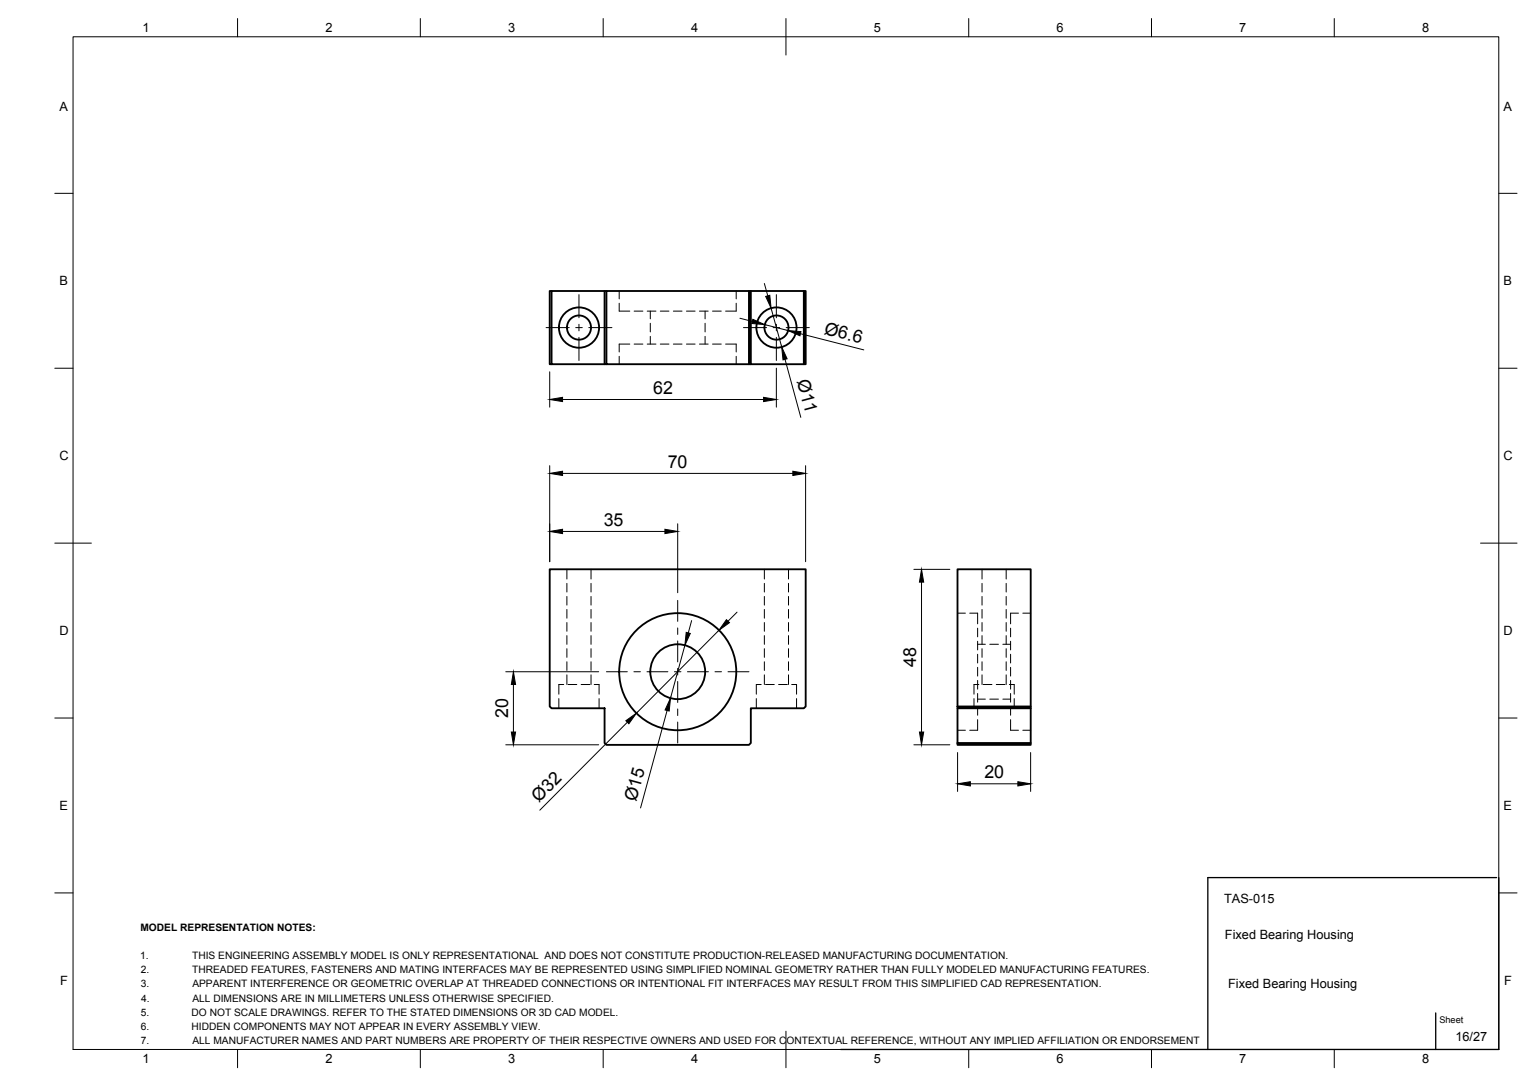
ISO-10303-21;
HEADER;
/* Generated by software containing ST-Developer
 * from STEP Tools, Inc. (www.steptools.com) 
 */

FILE_DESCRIPTION(
/* description */ ('STEP AP214'),
/* implementation_level */ '2;1');

FILE_NAME(
/* name */ 'Fixed Bearing Housing.step',
/* time_stamp */ '2026-11-15T14:49:54-08:00',
/* author */ (''),
/* organization */ (''),
/* preprocessor_version */ 'ST-DEVELOPER v20.2',
/* originating_system */ 'Autodesk Translation Framework v15.17.0.0',
/* authorisation */ '');

FILE_SCHEMA (('AUTOMOTIVE_DESIGN { 1 0 10303 214 3 1 1 }'));
ENDSEC;

DATA;
#10=MECHANICAL_DESIGN_GEOMETRIC_PRESENTATION_REPRESENTATION('',(#1109),#66721);
#1047=SHAPE_REPRESENTATION_RELATIONSHIP('SRR','None',#66907,#1078);
#1078=ADVANCED_BREP_SHAPE_REPRESENTATION('',(#1144),#66698);
#1109=STYLED_ITEM('',(#67095),#1144);
#1144=MANIFOLD_SOLID_BREP('Body1',#25675);
#1328=FACE_BOUND('',#4545,.T.);
#1329=FACE_BOUND('',#4549,.T.);
#1330=FACE_BOUND('',#4550,.T.);
#1331=FACE_BOUND('',#4554,.T.);
#1332=FACE_BOUND('',#4561,.T.);
#1333=FACE_BOUND('',#4563,.T.);
#1334=FACE_BOUND('',#4565,.T.);
#1335=FACE_BOUND('',#4567,.T.);
#1336=FACE_BOUND('',#4569,.T.);
#1337=FACE_BOUND('',#4571,.T.);
#1889=PLANE('',#27417);
#1890=PLANE('',#27418);
#1891=PLANE('',#27419);
#1892=PLANE('',#27420);
#1893=PLANE('',#27421);
#1894=PLANE('',#27422);
#1895=PLANE('',#27423);
#1896=PLANE('',#27424);
#1897=PLANE('',#27425);
#1898=PLANE('',#27426);
#1899=PLANE('',#27427);
#1900=PLANE('',#27428);
#1901=PLANE('',#27429);
#1902=PLANE('',#27430);
#1903=PLANE('',#27431);
#1904=PLANE('',#27432);
#1905=PLANE('',#27433);
#1906=PLANE('',#27434);
#2935=FACE_OUTER_BOUND('',#4537,.T.);
#2936=FACE_OUTER_BOUND('',#4538,.T.);
#2937=FACE_OUTER_BOUND('',#4539,.T.);
#2938=FACE_OUTER_BOUND('',#4540,.T.);
#2939=FACE_OUTER_BOUND('',#4541,.T.);
#2940=FACE_OUTER_BOUND('',#4542,.T.);
#2941=FACE_OUTER_BOUND('',#4543,.T.);
#2942=FACE_OUTER_BOUND('',#4544,.T.);
#2943=FACE_OUTER_BOUND('',#4546,.T.);
#2944=FACE_OUTER_BOUND('',#4547,.T.);
#2945=FACE_OUTER_BOUND('',#4548,.T.);
#2946=FACE_OUTER_BOUND('',#4551,.T.);
#2947=FACE_OUTER_BOUND('',#4552,.T.);
#2948=FACE_OUTER_BOUND('',#4553,.T.);
#2949=FACE_OUTER_BOUND('',#4555,.T.);
#2950=FACE_OUTER_BOUND('',#4556,.T.);
#2951=FACE_OUTER_BOUND('',#4557,.T.);
#2952=FACE_OUTER_BOUND('',#4558,.T.);
#2953=FACE_OUTER_BOUND('',#4559,.T.);
#2954=FACE_OUTER_BOUND('',#4560,.T.);
#2955=FACE_OUTER_BOUND('',#4562,.T.);
#2956=FACE_OUTER_BOUND('',#4564,.T.);
#2957=FACE_OUTER_BOUND('',#4566,.T.);
#2958=FACE_OUTER_BOUND('',#4568,.T.);
#2959=FACE_OUTER_BOUND('',#4570,.T.);
#4537=EDGE_LOOP('',(#20216,#20217,#20218,#20219));
#4538=EDGE_LOOP('',(#20220,#20221,#20222,#20223));
#4539=EDGE_LOOP('',(#20224,#20225,#20226,#20227));
#4540=EDGE_LOOP('',(#20228,#20229,#20230,#20231));
#4541=EDGE_LOOP('',(#20232,#20233,#20234,#20235));
#4542=EDGE_LOOP('',(#20236,#20237,#20238,#20239));
#4543=EDGE_LOOP('',(#20240,#20241,#20242,#20243));
#4544=EDGE_LOOP('',(#20244,#20245,#20246,#20247));
#4545=EDGE_LOOP('',(#20248));
#4546=EDGE_LOOP('',(#20249,#20250,#20251,#20252));
#4547=EDGE_LOOP('',(#20253,#20254,#20255,#20256));
#4548=EDGE_LOOP('',(#20257,#20258,#20259,#20260));
#4549=EDGE_LOOP('',(#20261));
#4550=EDGE_LOOP('',(#20262));
#4551=EDGE_LOOP('',(#20263,#20264,#20265,#20266));
#4552=EDGE_LOOP('',(#20267,#20268,#20269,#20270));
#4553=EDGE_LOOP('',(#20271,#20272,#20273,#20274));
#4554=EDGE_LOOP('',(#20275));
#4555=EDGE_LOOP('',(#20276,#20277,#20278,#20279));
#4556=EDGE_LOOP('',(#20280,#20281,#20282,#20283));
#4557=EDGE_LOOP('',(#20284,#20285,#20286,#20287));
#4558=EDGE_LOOP('',(#20288,#20289,#20290,#20291));
#4559=EDGE_LOOP('',(#20292,#20293,#20294,#20295));
#4560=EDGE_LOOP('',(#20296,#20297,#20298,#20299,#20300,#20301,#20302,#20303,
#20304,#20305,#20306,#20307));
#4561=EDGE_LOOP('',(#20308));
#4562=EDGE_LOOP('',(#20309,#20310,#20311,#20312,#20313,#20314,#20315,#20316,
#20317,#20318,#20319,#20320));
#4563=EDGE_LOOP('',(#20321));
#4564=EDGE_LOOP('',(#20322));
#4565=EDGE_LOOP('',(#20323));
#4566=EDGE_LOOP('',(#20324));
#4567=EDGE_LOOP('',(#20325));
#4568=EDGE_LOOP('',(#20326));
#4569=EDGE_LOOP('',(#20327));
#4570=EDGE_LOOP('',(#20328));
#4571=EDGE_LOOP('',(#20329));
#6589=LINE('',#40218,#8578);
#6590=LINE('',#40224,#8579);
#6591=LINE('',#40230,#8580);
#6592=LINE('',#40236,#8581);
#6593=LINE('',#40242,#8582);
#6594=LINE('',#40248,#8583);
#6595=LINE('',#40254,#8584);
#6596=LINE('',#40259,#8585);
#6597=LINE('',#40261,#8586);
#6598=LINE('',#40263,#8587);
#6599=LINE('',#40264,#8588);
#6600=LINE('',#40267,#8589);
#6601=LINE('',#40269,#8590);
#6602=LINE('',#40270,#8591);
#6603=LINE('',#40273,#8592);
#6604=LINE('',#40275,#8593);
#6605=LINE('',#40276,#8594);
#6606=LINE('',#40279,#8595);
#6607=LINE('',#40281,#8596);
#6608=LINE('',#40282,#8597);
#6609=LINE('',#40285,#8598);
#6610=LINE('',#40287,#8599);
#6611=LINE('',#40288,#8600);
#6612=LINE('',#40291,#8601);
#6613=LINE('',#40293,#8602);
#6614=LINE('',#40294,#8603);
#6615=LINE('',#40297,#8604);
#6616=LINE('',#40299,#8605);
#6617=LINE('',#40300,#8606);
#6618=LINE('',#40303,#8607);
#6619=LINE('',#40305,#8608);
#6620=LINE('',#40306,#8609);
#6621=LINE('',#40309,#8610);
#6622=LINE('',#40311,#8611);
#6623=LINE('',#40312,#8612);
#6624=LINE('',#40315,#8613);
#6625=LINE('',#40317,#8614);
#6626=LINE('',#40318,#8615);
#6627=LINE('',#40321,#8616);
#6628=LINE('',#40323,#8617);
#6629=LINE('',#40324,#8618);
#6630=LINE('',#40326,#8619);
#6631=LINE('',#40327,#8620);
#8578=VECTOR('',#32576,16.);
#8579=VECTOR('',#32583,7.5);
#8580=VECTOR('',#32590,16.);
#8581=VECTOR('',#32597,5.5);
#8582=VECTOR('',#32604,3.3);
#8583=VECTOR('',#32611,5.5);
#8584=VECTOR('',#32618,3.3);
#8585=VECTOR('',#32623,1000.);
#8586=VECTOR('',#32624,1000.);
#8587=VECTOR('',#32625,1000.);
#8588=VECTOR('',#32626,1000.);
#8589=VECTOR('',#32629,1000.);
#8590=VECTOR('',#32630,1000.);
#8591=VECTOR('',#32631,1000.);
#8592=VECTOR('',#32634,1000.);
#8593=VECTOR('',#32635,1000.);
#8594=VECTOR('',#32636,1000.);
#8595=VECTOR('',#32639,1000.);
#8596=VECTOR('',#32640,1000.);
#8597=VECTOR('',#32641,1000.);
#8598=VECTOR('',#32644,1000.);
#8599=VECTOR('',#32645,1000.);
#8600=VECTOR('',#32646,1000.);
#8601=VECTOR('',#32649,1000.);
#8602=VECTOR('',#32650,1000.);
#8603=VECTOR('',#32651,1000.);
#8604=VECTOR('',#32654,1000.);
#8605=VECTOR('',#32655,1000.);
#8606=VECTOR('',#32656,1000.);
#8607=VECTOR('',#32659,1000.);
#8608=VECTOR('',#32660,1000.);
#8609=VECTOR('',#32661,1000.);
#8610=VECTOR('',#32664,1000.);
#8611=VECTOR('',#32665,1000.);
#8612=VECTOR('',#32666,1000.);
#8613=VECTOR('',#32669,1000.);
#8614=VECTOR('',#32670,1000.);
#8615=VECTOR('',#32671,1000.);
#8616=VECTOR('',#32674,1000.);
#8617=VECTOR('',#32675,1000.);
#8618=VECTOR('',#32676,1000.);
#8619=VECTOR('',#32679,1000.);
#8620=VECTOR('',#32680,1000.);
#10044=CIRCLE('',#27397,16.);
#10045=CIRCLE('',#27398,16.);
#10046=CIRCLE('',#27400,7.5);
#10047=CIRCLE('',#27401,7.5);
#10048=CIRCLE('',#27403,16.);
#10049=CIRCLE('',#27404,16.);
#10050=CIRCLE('',#27406,5.5);
#10051=CIRCLE('',#27407,5.5);
#10052=CIRCLE('',#27409,3.29999999999999);
#10053=CIRCLE('',#27410,3.3);
#10054=CIRCLE('',#27412,5.5);
#10055=CIRCLE('',#27413,5.5);
#10056=CIRCLE('',#27415,3.29999999999999);
#10057=CIRCLE('',#27416,3.3);
#11835=VERTEX_POINT('',#40215);
#11836=VERTEX_POINT('',#40217);
#11837=VERTEX_POINT('',#40221);
#11838=VERTEX_POINT('',#40223);
#11839=VERTEX_POINT('',#40227);
#11840=VERTEX_POINT('',#40229);
#11841=VERTEX_POINT('',#40233);
#11842=VERTEX_POINT('',#40235);
#11843=VERTEX_POINT('',#40239);
#11844=VERTEX_POINT('',#40241);
#11845=VERTEX_POINT('',#40245);
#11846=VERTEX_POINT('',#40247);
#11847=VERTEX_POINT('',#40251);
#11848=VERTEX_POINT('',#40253);
#11849=VERTEX_POINT('',#40257);
#11850=VERTEX_POINT('',#40258);
#11851=VERTEX_POINT('',#40260);
#11852=VERTEX_POINT('',#40262);
#11853=VERTEX_POINT('',#40266);
#11854=VERTEX_POINT('',#40268);
#11855=VERTEX_POINT('',#40272);
#11856=VERTEX_POINT('',#40274);
#11857=VERTEX_POINT('',#40278);
#11858=VERTEX_POINT('',#40280);
#11859=VERTEX_POINT('',#40284);
#11860=VERTEX_POINT('',#40286);
#11861=VERTEX_POINT('',#40290);
#11862=VERTEX_POINT('',#40292);
#11863=VERTEX_POINT('',#40296);
#11864=VERTEX_POINT('',#40298);
#11865=VERTEX_POINT('',#40302);
#11866=VERTEX_POINT('',#40304);
#11867=VERTEX_POINT('',#40308);
#11868=VERTEX_POINT('',#40310);
#11869=VERTEX_POINT('',#40314);
#11870=VERTEX_POINT('',#40316);
#11871=VERTEX_POINT('',#40320);
#11872=VERTEX_POINT('',#40322);
#14801=EDGE_CURVE('',#11835,#11835,#10044,.T.);
#14802=EDGE_CURVE('',#11835,#11836,#6589,.T.);
#14803=EDGE_CURVE('',#11836,#11836,#10045,.T.);
#14804=EDGE_CURVE('',#11837,#11837,#10046,.T.);
#14805=EDGE_CURVE('',#11837,#11838,#6590,.T.);
#14806=EDGE_CURVE('',#11838,#11838,#10047,.T.);
#14807=EDGE_CURVE('',#11839,#11839,#10048,.T.);
#14808=EDGE_CURVE('',#11839,#11840,#6591,.T.);
#14809=EDGE_CURVE('',#11840,#11840,#10049,.T.);
#14810=EDGE_CURVE('',#11841,#11841,#10050,.T.);
#14811=EDGE_CURVE('',#11841,#11842,#6592,.T.);
#14812=EDGE_CURVE('',#11842,#11842,#10051,.T.);
#14813=EDGE_CURVE('',#11843,#11843,#10052,.T.);
#14814=EDGE_CURVE('',#11843,#11844,#6593,.T.);
#14815=EDGE_CURVE('',#11844,#11844,#10053,.T.);
#14816=EDGE_CURVE('',#11845,#11845,#10054,.T.);
#14817=EDGE_CURVE('',#11845,#11846,#6594,.T.);
#14818=EDGE_CURVE('',#11846,#11846,#10055,.T.);
#14819=EDGE_CURVE('',#11847,#11847,#10056,.T.);
#14820=EDGE_CURVE('',#11847,#11848,#6595,.T.);
#14821=EDGE_CURVE('',#11848,#11848,#10057,.T.);
#14822=EDGE_CURVE('',#11849,#11850,#6596,.T.);
#14823=EDGE_CURVE('',#11851,#11850,#6597,.T.);
#14824=EDGE_CURVE('',#11852,#11851,#6598,.T.);
#14825=EDGE_CURVE('',#11852,#11849,#6599,.T.);
#14826=EDGE_CURVE('',#11850,#11853,#6600,.T.);
#14827=EDGE_CURVE('',#11854,#11853,#6601,.T.);
#14828=EDGE_CURVE('',#11851,#11854,#6602,.T.);
#14829=EDGE_CURVE('',#11853,#11855,#6603,.T.);
#14830=EDGE_CURVE('',#11856,#11855,#6604,.T.);
#14831=EDGE_CURVE('',#11854,#11856,#6605,.T.);
#14832=EDGE_CURVE('',#11855,#11857,#6606,.T.);
#14833=EDGE_CURVE('',#11858,#11857,#6607,.T.);
#14834=EDGE_CURVE('',#11856,#11858,#6608,.T.);
#14835=EDGE_CURVE('',#11857,#11859,#6609,.T.);
#14836=EDGE_CURVE('',#11860,#11859,#6610,.T.);
#14837=EDGE_CURVE('',#11858,#11860,#6611,.T.);
#14838=EDGE_CURVE('',#11859,#11861,#6612,.T.);
#14839=EDGE_CURVE('',#11862,#11861,#6613,.T.);
#14840=EDGE_CURVE('',#11860,#11862,#6614,.T.);
#14841=EDGE_CURVE('',#11861,#11863,#6615,.T.);
#14842=EDGE_CURVE('',#11864,#11863,#6616,.T.);
#14843=EDGE_CURVE('',#11862,#11864,#6617,.T.);
#14844=EDGE_CURVE('',#11863,#11865,#6618,.T.);
#14845=EDGE_CURVE('',#11866,#11865,#6619,.T.);
#14846=EDGE_CURVE('',#11864,#11866,#6620,.T.);
#14847=EDGE_CURVE('',#11865,#11867,#6621,.T.);
#14848=EDGE_CURVE('',#11868,#11867,#6622,.T.);
#14849=EDGE_CURVE('',#11866,#11868,#6623,.T.);
#14850=EDGE_CURVE('',#11867,#11869,#6624,.T.);
#14851=EDGE_CURVE('',#11870,#11869,#6625,.T.);
#14852=EDGE_CURVE('',#11868,#11870,#6626,.T.);
#14853=EDGE_CURVE('',#11869,#11871,#6627,.T.);
#14854=EDGE_CURVE('',#11872,#11871,#6628,.T.);
#14855=EDGE_CURVE('',#11870,#11872,#6629,.T.);
#14856=EDGE_CURVE('',#11871,#11849,#6630,.T.);
#14857=EDGE_CURVE('',#11872,#11852,#6631,.T.);
#20216=ORIENTED_EDGE('',*,*,#14801,.F.);
#20217=ORIENTED_EDGE('',*,*,#14802,.T.);
#20218=ORIENTED_EDGE('',*,*,#14803,.T.);
#20219=ORIENTED_EDGE('',*,*,#14802,.F.);
#20220=ORIENTED_EDGE('',*,*,#14804,.F.);
#20221=ORIENTED_EDGE('',*,*,#14805,.T.);
#20222=ORIENTED_EDGE('',*,*,#14806,.T.);
#20223=ORIENTED_EDGE('',*,*,#14805,.F.);
#20224=ORIENTED_EDGE('',*,*,#14807,.F.);
#20225=ORIENTED_EDGE('',*,*,#14808,.T.);
#20226=ORIENTED_EDGE('',*,*,#14809,.T.);
#20227=ORIENTED_EDGE('',*,*,#14808,.F.);
#20228=ORIENTED_EDGE('',*,*,#14810,.F.);
#20229=ORIENTED_EDGE('',*,*,#14811,.T.);
#20230=ORIENTED_EDGE('',*,*,#14812,.T.);
#20231=ORIENTED_EDGE('',*,*,#14811,.F.);
#20232=ORIENTED_EDGE('',*,*,#14813,.F.);
#20233=ORIENTED_EDGE('',*,*,#14814,.T.);
#20234=ORIENTED_EDGE('',*,*,#14815,.T.);
#20235=ORIENTED_EDGE('',*,*,#14814,.F.);
#20236=ORIENTED_EDGE('',*,*,#14816,.F.);
#20237=ORIENTED_EDGE('',*,*,#14817,.T.);
#20238=ORIENTED_EDGE('',*,*,#14818,.T.);
#20239=ORIENTED_EDGE('',*,*,#14817,.F.);
#20240=ORIENTED_EDGE('',*,*,#14819,.F.);
#20241=ORIENTED_EDGE('',*,*,#14820,.T.);
#20242=ORIENTED_EDGE('',*,*,#14821,.T.);
#20243=ORIENTED_EDGE('',*,*,#14820,.F.);
#20244=ORIENTED_EDGE('',*,*,#14822,.T.);
#20245=ORIENTED_EDGE('',*,*,#14823,.F.);
#20246=ORIENTED_EDGE('',*,*,#14824,.F.);
#20247=ORIENTED_EDGE('',*,*,#14825,.T.);
#20248=ORIENTED_EDGE('',*,*,#14818,.F.);
#20249=ORIENTED_EDGE('',*,*,#14826,.T.);
#20250=ORIENTED_EDGE('',*,*,#14827,.F.);
#20251=ORIENTED_EDGE('',*,*,#14828,.F.);
#20252=ORIENTED_EDGE('',*,*,#14823,.T.);
#20253=ORIENTED_EDGE('',*,*,#14829,.T.);
#20254=ORIENTED_EDGE('',*,*,#14830,.F.);
#20255=ORIENTED_EDGE('',*,*,#14831,.F.);
#20256=ORIENTED_EDGE('',*,*,#14827,.T.);
#20257=ORIENTED_EDGE('',*,*,#14832,.T.);
#20258=ORIENTED_EDGE('',*,*,#14833,.F.);
#20259=ORIENTED_EDGE('',*,*,#14834,.F.);
#20260=ORIENTED_EDGE('',*,*,#14830,.T.);
#20261=ORIENTED_EDGE('',*,*,#14813,.T.);
#20262=ORIENTED_EDGE('',*,*,#14819,.T.);
#20263=ORIENTED_EDGE('',*,*,#14835,.T.);
#20264=ORIENTED_EDGE('',*,*,#14836,.F.);
#20265=ORIENTED_EDGE('',*,*,#14837,.F.);
#20266=ORIENTED_EDGE('',*,*,#14833,.T.);
#20267=ORIENTED_EDGE('',*,*,#14838,.T.);
#20268=ORIENTED_EDGE('',*,*,#14839,.F.);
#20269=ORIENTED_EDGE('',*,*,#14840,.F.);
#20270=ORIENTED_EDGE('',*,*,#14836,.T.);
#20271=ORIENTED_EDGE('',*,*,#14841,.T.);
#20272=ORIENTED_EDGE('',*,*,#14842,.F.);
#20273=ORIENTED_EDGE('',*,*,#14843,.F.);
#20274=ORIENTED_EDGE('',*,*,#14839,.T.);
#20275=ORIENTED_EDGE('',*,*,#14812,.F.);
#20276=ORIENTED_EDGE('',*,*,#14844,.T.);
#20277=ORIENTED_EDGE('',*,*,#14845,.F.);
#20278=ORIENTED_EDGE('',*,*,#14846,.F.);
#20279=ORIENTED_EDGE('',*,*,#14842,.T.);
#20280=ORIENTED_EDGE('',*,*,#14847,.T.);
#20281=ORIENTED_EDGE('',*,*,#14848,.F.);
#20282=ORIENTED_EDGE('',*,*,#14849,.F.);
#20283=ORIENTED_EDGE('',*,*,#14845,.T.);
#20284=ORIENTED_EDGE('',*,*,#14850,.T.);
#20285=ORIENTED_EDGE('',*,*,#14851,.F.);
#20286=ORIENTED_EDGE('',*,*,#14852,.F.);
#20287=ORIENTED_EDGE('',*,*,#14848,.T.);
#20288=ORIENTED_EDGE('',*,*,#14853,.T.);
#20289=ORIENTED_EDGE('',*,*,#14854,.F.);
#20290=ORIENTED_EDGE('',*,*,#14855,.F.);
#20291=ORIENTED_EDGE('',*,*,#14851,.T.);
#20292=ORIENTED_EDGE('',*,*,#14856,.T.);
#20293=ORIENTED_EDGE('',*,*,#14825,.F.);
#20294=ORIENTED_EDGE('',*,*,#14857,.F.);
#20295=ORIENTED_EDGE('',*,*,#14854,.T.);
#20296=ORIENTED_EDGE('',*,*,#14824,.T.);
#20297=ORIENTED_EDGE('',*,*,#14828,.T.);
#20298=ORIENTED_EDGE('',*,*,#14831,.T.);
#20299=ORIENTED_EDGE('',*,*,#14834,.T.);
#20300=ORIENTED_EDGE('',*,*,#14837,.T.);
#20301=ORIENTED_EDGE('',*,*,#14840,.T.);
#20302=ORIENTED_EDGE('',*,*,#14843,.T.);
#20303=ORIENTED_EDGE('',*,*,#14846,.T.);
#20304=ORIENTED_EDGE('',*,*,#14849,.T.);
#20305=ORIENTED_EDGE('',*,*,#14852,.T.);
#20306=ORIENTED_EDGE('',*,*,#14855,.T.);
#20307=ORIENTED_EDGE('',*,*,#14857,.T.);
#20308=ORIENTED_EDGE('',*,*,#14803,.F.);
#20309=ORIENTED_EDGE('',*,*,#14822,.F.);
#20310=ORIENTED_EDGE('',*,*,#14856,.F.);
#20311=ORIENTED_EDGE('',*,*,#14853,.F.);
#20312=ORIENTED_EDGE('',*,*,#14850,.F.);
#20313=ORIENTED_EDGE('',*,*,#14847,.F.);
#20314=ORIENTED_EDGE('',*,*,#14844,.F.);
#20315=ORIENTED_EDGE('',*,*,#14841,.F.);
#20316=ORIENTED_EDGE('',*,*,#14838,.F.);
#20317=ORIENTED_EDGE('',*,*,#14835,.F.);
#20318=ORIENTED_EDGE('',*,*,#14832,.F.);
#20319=ORIENTED_EDGE('',*,*,#14829,.F.);
#20320=ORIENTED_EDGE('',*,*,#14826,.F.);
#20321=ORIENTED_EDGE('',*,*,#14807,.T.);
#20322=ORIENTED_EDGE('',*,*,#14816,.T.);
#20323=ORIENTED_EDGE('',*,*,#14821,.F.);
#20324=ORIENTED_EDGE('',*,*,#14810,.T.);
#20325=ORIENTED_EDGE('',*,*,#14815,.F.);
#20326=ORIENTED_EDGE('',*,*,#14809,.F.);
#20327=ORIENTED_EDGE('',*,*,#14804,.T.);
#20328=ORIENTED_EDGE('',*,*,#14801,.T.);
#20329=ORIENTED_EDGE('',*,*,#14806,.F.);
#24042=CYLINDRICAL_SURFACE('',#27396,16.);
#24043=CYLINDRICAL_SURFACE('',#27399,7.5);
#24044=CYLINDRICAL_SURFACE('',#27402,16.);
#24045=CYLINDRICAL_SURFACE('',#27405,5.5);
#24046=CYLINDRICAL_SURFACE('',#27408,3.3);
#24047=CYLINDRICAL_SURFACE('',#27411,5.5);
#24048=CYLINDRICAL_SURFACE('',#27414,3.3);
#24888=ADVANCED_FACE('',(#2935),#24042,.F.);
#24889=ADVANCED_FACE('',(#2936),#24043,.F.);
#24890=ADVANCED_FACE('',(#2937),#24044,.F.);
#24891=ADVANCED_FACE('',(#2938),#24045,.F.);
#24892=ADVANCED_FACE('',(#2939),#24046,.F.);
#24893=ADVANCED_FACE('',(#2940),#24047,.F.);
#24894=ADVANCED_FACE('',(#2941),#24048,.F.);
#24895=ADVANCED_FACE('',(#2942,#1328),#1889,.F.);
#24896=ADVANCED_FACE('',(#2943),#1890,.F.);
#24897=ADVANCED_FACE('',(#2944),#1891,.F.);
#24898=ADVANCED_FACE('',(#2945,#1329,#1330),#1892,.F.);
#24899=ADVANCED_FACE('',(#2946),#1893,.F.);
#24900=ADVANCED_FACE('',(#2947),#1894,.F.);
#24901=ADVANCED_FACE('',(#2948,#1331),#1895,.F.);
#24902=ADVANCED_FACE('',(#2949),#1896,.F.);
#24903=ADVANCED_FACE('',(#2950),#1897,.F.);
#24904=ADVANCED_FACE('',(#2951),#1898,.F.);
#24905=ADVANCED_FACE('',(#2952),#1899,.F.);
#24906=ADVANCED_FACE('',(#2953),#1900,.F.);
#24907=ADVANCED_FACE('',(#2954,#1332),#1901,.T.);
#24908=ADVANCED_FACE('',(#2955,#1333),#1902,.F.);
#24909=ADVANCED_FACE('',(#2956,#1334),#1903,.F.);
#24910=ADVANCED_FACE('',(#2957,#1335),#1904,.F.);
#24911=ADVANCED_FACE('',(#2958,#1336),#1905,.F.);
#24912=ADVANCED_FACE('',(#2959,#1337),#1906,.F.);
#25675=CLOSED_SHELL('',(#24888,#24889,#24890,#24891,#24892,#24893,#24894,
#24895,#24896,#24897,#24898,#24899,#24900,#24901,#24902,#24903,#24904,#24905,
#24906,#24907,#24908,#24909,#24910,#24911,#24912));
#27395=AXIS2_PLACEMENT_3D('',#40213,#32570,#32571);
#27396=AXIS2_PLACEMENT_3D('',#40214,#32572,#32573);
#27397=AXIS2_PLACEMENT_3D('',#40216,#32574,#32575);
#27398=AXIS2_PLACEMENT_3D('',#40219,#32577,#32578);
#27399=AXIS2_PLACEMENT_3D('',#40220,#32579,#32580);
#27400=AXIS2_PLACEMENT_3D('',#40222,#32581,#32582);
#27401=AXIS2_PLACEMENT_3D('',#40225,#32584,#32585);
#27402=AXIS2_PLACEMENT_3D('',#40226,#32586,#32587);
#27403=AXIS2_PLACEMENT_3D('',#40228,#32588,#32589);
#27404=AXIS2_PLACEMENT_3D('',#40231,#32591,#32592);
#27405=AXIS2_PLACEMENT_3D('',#40232,#32593,#32594);
#27406=AXIS2_PLACEMENT_3D('',#40234,#32595,#32596);
#27407=AXIS2_PLACEMENT_3D('',#40237,#32598,#32599);
#27408=AXIS2_PLACEMENT_3D('',#40238,#32600,#32601);
#27409=AXIS2_PLACEMENT_3D('',#40240,#32602,#32603);
#27410=AXIS2_PLACEMENT_3D('',#40243,#32605,#32606);
#27411=AXIS2_PLACEMENT_3D('',#40244,#32607,#32608);
#27412=AXIS2_PLACEMENT_3D('',#40246,#32609,#32610);
#27413=AXIS2_PLACEMENT_3D('',#40249,#32612,#32613);
#27414=AXIS2_PLACEMENT_3D('',#40250,#32614,#32615);
#27415=AXIS2_PLACEMENT_3D('',#40252,#32616,#32617);
#27416=AXIS2_PLACEMENT_3D('',#40255,#32619,#32620);
#27417=AXIS2_PLACEMENT_3D('',#40256,#32621,#32622);
#27418=AXIS2_PLACEMENT_3D('',#40265,#32627,#32628);
#27419=AXIS2_PLACEMENT_3D('',#40271,#32632,#32633);
#27420=AXIS2_PLACEMENT_3D('',#40277,#32637,#32638);
#27421=AXIS2_PLACEMENT_3D('',#40283,#32642,#32643);
#27422=AXIS2_PLACEMENT_3D('',#40289,#32647,#32648);
#27423=AXIS2_PLACEMENT_3D('',#40295,#32652,#32653);
#27424=AXIS2_PLACEMENT_3D('',#40301,#32657,#32658);
#27425=AXIS2_PLACEMENT_3D('',#40307,#32662,#32663);
#27426=AXIS2_PLACEMENT_3D('',#40313,#32667,#32668);
#27427=AXIS2_PLACEMENT_3D('',#40319,#32672,#32673);
#27428=AXIS2_PLACEMENT_3D('',#40325,#32677,#32678);
#27429=AXIS2_PLACEMENT_3D('',#40328,#32681,#32682);
#27430=AXIS2_PLACEMENT_3D('',#40329,#32683,#32684);
#27431=AXIS2_PLACEMENT_3D('',#40330,#32685,#32686);
#27432=AXIS2_PLACEMENT_3D('',#40331,#32687,#32688);
#27433=AXIS2_PLACEMENT_3D('',#40332,#32689,#32690);
#27434=AXIS2_PLACEMENT_3D('',#40333,#32691,#32692);
#32570=DIRECTION('axis',(0.,0.,1.));
#32571=DIRECTION('refdir',(1.,0.,0.));
#32572=DIRECTION('center_axis',(1.,1.73472347597681E-16,0.));
#32573=DIRECTION('ref_axis',(-1.73472347597681E-16,1.,0.));
#32574=DIRECTION('center_axis',(1.,1.73472347597681E-16,0.));
#32575=DIRECTION('ref_axis',(-1.73472347597681E-16,1.,0.));
#32576=DIRECTION('',(1.,1.73472347597681E-16,0.));
#32577=DIRECTION('center_axis',(1.,1.73472347597681E-16,0.));
#32578=DIRECTION('ref_axis',(-1.73472347597681E-16,1.,0.));
#32579=DIRECTION('center_axis',(1.,1.73472347597681E-16,0.));
#32580=DIRECTION('ref_axis',(-1.73472347597681E-16,1.,0.));
#32581=DIRECTION('center_axis',(1.,1.73472347597681E-16,0.));
#32582=DIRECTION('ref_axis',(-1.73472347597681E-16,1.,0.));
#32583=DIRECTION('',(1.,1.73472347597681E-16,0.));
#32584=DIRECTION('center_axis',(1.,1.73472347597681E-16,0.));
#32585=DIRECTION('ref_axis',(-1.73472347597681E-16,1.,0.));
#32586=DIRECTION('center_axis',(1.,1.73472347597681E-16,0.));
#32587=DIRECTION('ref_axis',(-1.73472347597681E-16,1.,0.));
#32588=DIRECTION('center_axis',(1.,1.73472347597681E-16,0.));
#32589=DIRECTION('ref_axis',(-1.73472347597681E-16,1.,0.));
#32590=DIRECTION('',(1.,1.73472347597681E-16,0.));
#32591=DIRECTION('center_axis',(1.,1.73472347597681E-16,0.));
#32592=DIRECTION('ref_axis',(-1.73472347597681E-16,1.,0.));
#32593=DIRECTION('center_axis',(0.,1.,0.));
#32594=DIRECTION('ref_axis',(0.,0.,1.));
#32595=DIRECTION('center_axis',(0.,1.,0.));
#32596=DIRECTION('ref_axis',(0.,0.,1.));
#32597=DIRECTION('',(0.,1.,0.));
#32598=DIRECTION('center_axis',(0.,1.,0.));
#32599=DIRECTION('ref_axis',(0.,0.,1.));
#32600=DIRECTION('center_axis',(0.,1.,0.));
#32601=DIRECTION('ref_axis',(0.,0.,1.));
#32602=DIRECTION('center_axis',(0.,1.,0.));
#32603=DIRECTION('ref_axis',(0.,0.,1.));
#32604=DIRECTION('',(0.,1.,0.));
#32605=DIRECTION('center_axis',(0.,1.,0.));
#32606=DIRECTION('ref_axis',(0.,0.,1.));
#32607=DIRECTION('center_axis',(0.,1.,0.));
#32608=DIRECTION('ref_axis',(0.,0.,1.));
#32609=DIRECTION('center_axis',(0.,1.,0.));
#32610=DIRECTION('ref_axis',(0.,0.,1.));
#32611=DIRECTION('',(0.,1.,0.));
#32612=DIRECTION('center_axis',(0.,1.,0.));
#32613=DIRECTION('ref_axis',(0.,0.,1.));
#32614=DIRECTION('center_axis',(0.,1.,0.));
#32615=DIRECTION('ref_axis',(0.,0.,1.));
#32616=DIRECTION('center_axis',(0.,1.,0.));
#32617=DIRECTION('ref_axis',(0.,0.,1.));
#32618=DIRECTION('',(0.,1.,0.));
#32619=DIRECTION('center_axis',(0.,1.,0.));
#32620=DIRECTION('ref_axis',(0.,0.,1.));
#32621=DIRECTION('center_axis',(0.,-1.,-4.78544407166016E-16));
#32622=DIRECTION('ref_axis',(0.,4.78544407166016E-16,-1.));
#32623=DIRECTION('',(0.,-4.78544407166016E-16,1.));
#32624=DIRECTION('',(-1.,0.,0.));
#32625=DIRECTION('',(0.,-4.78544407166016E-16,1.));
#32626=DIRECTION('',(-1.,0.,0.));
#32627=DIRECTION('center_axis',(0.,-0.707106781186528,-0.707106781186567));
#32628=DIRECTION('ref_axis',(0.,0.707106781186567,-0.707106781186528));
#32629=DIRECTION('',(0.,-0.707106781186567,0.707106781186528));
#32630=DIRECTION('',(-1.,0.,0.));
#32631=DIRECTION('',(0.,-0.707106781186567,0.707106781186528));
#32632=DIRECTION('center_axis',(0.,3.70074341541719E-16,-1.));
#32633=DIRECTION('ref_axis',(0.,1.,3.70074341541719E-16));
#32634=DIRECTION('',(0.,-1.,-3.70074341541719E-16));
#32635=DIRECTION('',(-1.,0.,0.));
#32636=DIRECTION('',(0.,-1.,-3.70074341541719E-16));
#32637=DIRECTION('center_axis',(0.,1.,3.11362923006336E-16));
#32638=DIRECTION('ref_axis',(0.,-3.11362923006336E-16,1.));
#32639=DIRECTION('',(0.,3.11362923006336E-16,-1.));
#32640=DIRECTION('',(-1.,0.,0.));
#32641=DIRECTION('',(0.,3.11362923006336E-16,-1.));
#32642=DIRECTION('center_axis',(0.,-5.55111512312579E-16,1.));
#32643=DIRECTION('ref_axis',(0.,-1.,-5.55111512312579E-16));
#32644=DIRECTION('',(0.,1.,5.55111512312579E-16));
#32645=DIRECTION('',(-1.,0.,0.));
#32646=DIRECTION('',(0.,1.,5.55111512312579E-16));
#32647=DIRECTION('center_axis',(0.,-0.707106781186538,0.707106781186557));
#32648=DIRECTION('ref_axis',(0.,-0.707106781186557,-0.707106781186538));
#32649=DIRECTION('',(0.,0.707106781186557,0.707106781186538));
#32650=DIRECTION('',(-1.,0.,0.));
#32651=DIRECTION('',(0.,0.707106781186557,0.707106781186538));
#32652=DIRECTION('center_axis',(0.,-1.,-4.78544407166016E-16));
#32653=DIRECTION('ref_axis',(0.,4.78544407166016E-16,-1.));
#32654=DIRECTION('',(0.,-4.78544407166016E-16,1.));
#32655=DIRECTION('',(-1.,0.,0.));
#32656=DIRECTION('',(0.,-4.78544407166016E-16,1.));
#32657=DIRECTION('center_axis',(0.,0.,1.));
#32658=DIRECTION('ref_axis',(1.,0.,0.));
#32659=DIRECTION('',(0.,1.,0.));
#32660=DIRECTION('',(-1.,0.,0.));
#32661=DIRECTION('',(0.,1.,0.));
#32662=DIRECTION('center_axis',(0.,-0.707106781186548,0.707106781186548));
#32663=DIRECTION('ref_axis',(0.,-0.707106781186548,-0.707106781186548));
#32664=DIRECTION('',(0.,0.707106781186547,0.707106781186547));
#32665=DIRECTION('',(-1.,0.,0.));
#32666=DIRECTION('',(0.,0.707106781186547,0.707106781186547));
#32667=DIRECTION('center_axis',(0.,-1.,1.77920356510442E-16));
#32668=DIRECTION('ref_axis',(0.,-1.77920356510442E-16,-1.));
#32669=DIRECTION('',(0.,1.77920356510442E-16,1.));
#32670=DIRECTION('',(-1.,0.,0.));
#32671=DIRECTION('',(0.,1.77920356510442E-16,1.));
#32672=DIRECTION('center_axis',(0.,-0.707106781186548,-0.707106781186548));
#32673=DIRECTION('ref_axis',(0.,0.707106781186548,-0.707106781186548));
#32674=DIRECTION('',(0.,-0.707106781186547,0.707106781186547));
#32675=DIRECTION('',(-1.,0.,0.));
#32676=DIRECTION('',(0.,-0.707106781186547,0.707106781186547));
#32677=DIRECTION('center_axis',(0.,3.65204942310907E-16,-1.));
#32678=DIRECTION('ref_axis',(0.,1.,3.65204942310907E-16));
#32679=DIRECTION('',(0.,-1.,-3.65204942310907E-16));
#32680=DIRECTION('',(0.,-1.,-3.65204942310907E-16));
#32681=DIRECTION('center_axis',(1.,0.,0.));
#32682=DIRECTION('ref_axis',(0.,0.,-1.));
#32683=DIRECTION('center_axis',(1.,0.,0.));
#32684=DIRECTION('ref_axis',(0.,0.,-1.));
#32685=DIRECTION('center_axis',(0.,-1.,0.));
#32686=DIRECTION('ref_axis',(0.,0.,-1.));
#32687=DIRECTION('center_axis',(0.,-1.,0.));
#32688=DIRECTION('ref_axis',(0.,0.,-1.));
#32689=DIRECTION('center_axis',(1.,1.73472347597681E-16,0.));
#32690=DIRECTION('ref_axis',(-1.73472347597681E-16,1.,0.));
#32691=DIRECTION('center_axis',(-1.,-1.73472347597681E-16,0.));
#32692=DIRECTION('ref_axis',(1.73472347597681E-16,-1.,0.));
#40213=CARTESIAN_POINT('',(0.,0.,0.));
#40214=CARTESIAN_POINT('Origin',(20.,28.,0.));
#40215=CARTESIAN_POINT('',(14.5,12.,-1.95943487863577E-15));
#40216=CARTESIAN_POINT('Origin',(14.5,28.,0.));
#40217=CARTESIAN_POINT('',(20.,12.,-1.95943487863577E-15));
#40218=CARTESIAN_POINT('',(20.,12.,-1.95943487863577E-15));
#40219=CARTESIAN_POINT('Origin',(20.,28.,0.));
#40220=CARTESIAN_POINT('Origin',(20.,28.,0.));
#40221=CARTESIAN_POINT('',(5.5,20.5,-9.18485099360515E-16));
#40222=CARTESIAN_POINT('Origin',(5.5,28.,0.));
#40223=CARTESIAN_POINT('',(14.5,20.5,-9.18485099360515E-16));
#40224=CARTESIAN_POINT('',(20.,20.5,-9.18485099360515E-16));
#40225=CARTESIAN_POINT('Origin',(14.5,28.,0.));
#40226=CARTESIAN_POINT('Origin',(20.,28.,0.));
#40227=CARTESIAN_POINT('',(6.66133814775094E-15,12.,-1.95943487863577E-15));
#40228=CARTESIAN_POINT('Origin',(3.46944695195361E-15,28.,0.));
#40229=CARTESIAN_POINT('',(5.50000000000001,12.,-1.95943487863577E-15));
#40230=CARTESIAN_POINT('',(20.,12.,-1.95943487863577E-15));
#40231=CARTESIAN_POINT('Origin',(5.5,28.,0.));
#40232=CARTESIAN_POINT('Origin',(10.,38.,-27.));
#40233=CARTESIAN_POINT('',(10.,31.5,-32.5));
#40234=CARTESIAN_POINT('Origin',(10.,31.5,-27.));
#40235=CARTESIAN_POINT('',(10.,38.,-32.5));
#40236=CARTESIAN_POINT('',(10.,38.,-32.5));
#40237=CARTESIAN_POINT('Origin',(10.,38.,-27.));
#40238=CARTESIAN_POINT('Origin',(10.,38.,-27.));
#40239=CARTESIAN_POINT('',(10.,0.,-30.3));
#40240=CARTESIAN_POINT('Origin',(10.,0.,-27.));
#40241=CARTESIAN_POINT('',(10.,31.5,-30.3));
#40242=CARTESIAN_POINT('',(10.,38.,-30.3));
#40243=CARTESIAN_POINT('Origin',(10.,31.5,-27.));
#40244=CARTESIAN_POINT('Origin',(10.,38.,27.));
#40245=CARTESIAN_POINT('',(9.99999999999999,31.5,21.5));
#40246=CARTESIAN_POINT('Origin',(10.,31.5,27.));
#40247=CARTESIAN_POINT('',(9.99999999999999,38.,21.5));
#40248=CARTESIAN_POINT('',(9.99999999999999,38.,21.5));
#40249=CARTESIAN_POINT('Origin',(10.,38.,27.));
#40250=CARTESIAN_POINT('Origin',(10.,38.,27.));
#40251=CARTESIAN_POINT('',(10.,0.,23.7));
#40252=CARTESIAN_POINT('Origin',(10.,0.,27.));
#40253=CARTESIAN_POINT('',(10.,31.5,23.7));
#40254=CARTESIAN_POINT('',(10.,38.,23.7));
#40255=CARTESIAN_POINT('Origin',(10.,31.5,27.));
#40256=CARTESIAN_POINT('Origin',(20.,38.,20.));
#40257=CARTESIAN_POINT('',(0.,38.,20.));
#40258=CARTESIAN_POINT('',(0.,38.,34.5));
#40259=CARTESIAN_POINT('',(0.,38.,20.));
#40260=CARTESIAN_POINT('',(20.,38.,34.5));
#40261=CARTESIAN_POINT('',(20.,38.,34.5));
#40262=CARTESIAN_POINT('',(20.,38.,20.));
#40263=CARTESIAN_POINT('',(20.,38.,20.));
#40264=CARTESIAN_POINT('',(20.,38.,20.));
#40265=CARTESIAN_POINT('Origin',(20.,38.,34.5));
#40266=CARTESIAN_POINT('',(0.,37.5,35.));
#40267=CARTESIAN_POINT('',(0.,38.,34.5));
#40268=CARTESIAN_POINT('',(20.,37.5,35.));
#40269=CARTESIAN_POINT('',(20.,37.5,35.));
#40270=CARTESIAN_POINT('',(20.,38.,34.5));
#40271=CARTESIAN_POINT('Origin',(20.,37.5,35.));
#40272=CARTESIAN_POINT('',(0.,-7.70371977754894E-31,35.));
#40273=CARTESIAN_POINT('',(0.,37.5,35.));
#40274=CARTESIAN_POINT('',(20.,-7.70371977754894E-31,35.));
#40275=CARTESIAN_POINT('',(20.,-7.70371977754894E-31,35.));
#40276=CARTESIAN_POINT('',(20.,37.5,35.));
#40277=CARTESIAN_POINT('Origin',(20.,-7.70371977754894E-31,35.));
#40278=CARTESIAN_POINT('',(0.,2.17954046104435E-14,-35.));
#40279=CARTESIAN_POINT('',(0.,-7.70371977754894E-31,35.));
#40280=CARTESIAN_POINT('',(20.,2.17954046104435E-14,-35.));
#40281=CARTESIAN_POINT('',(20.,2.17954046104435E-14,-35.));
#40282=CARTESIAN_POINT('',(20.,-7.70371977754894E-31,35.));
#40283=CARTESIAN_POINT('Origin',(20.,37.5,-35.));
#40284=CARTESIAN_POINT('',(0.,37.5,-35.));
#40285=CARTESIAN_POINT('',(0.,37.5,-35.));
#40286=CARTESIAN_POINT('',(20.,37.5,-35.));
#40287=CARTESIAN_POINT('',(20.,37.5,-35.));
#40288=CARTESIAN_POINT('',(20.,37.5,-35.));
#40289=CARTESIAN_POINT('Origin',(20.,38.,-34.5));
#40290=CARTESIAN_POINT('',(0.,38.,-34.5));
#40291=CARTESIAN_POINT('',(0.,38.,-34.5));
#40292=CARTESIAN_POINT('',(20.,38.,-34.5));
#40293=CARTESIAN_POINT('',(20.,38.,-34.5));
#40294=CARTESIAN_POINT('',(20.,38.,-34.5));
#40295=CARTESIAN_POINT('Origin',(20.,38.,-20.));
#40296=CARTESIAN_POINT('',(0.,38.,-20.));
#40297=CARTESIAN_POINT('',(0.,38.,-20.));
#40298=CARTESIAN_POINT('',(20.,38.,-20.));
#40299=CARTESIAN_POINT('',(20.,38.,-20.));
#40300=CARTESIAN_POINT('',(20.,38.,-20.));
#40301=CARTESIAN_POINT('Origin',(20.,47.5,-20.));
#40302=CARTESIAN_POINT('',(0.,47.5,-20.));
#40303=CARTESIAN_POINT('',(0.,47.5,-20.));
#40304=CARTESIAN_POINT('',(20.,47.5,-20.));
#40305=CARTESIAN_POINT('',(20.,47.5,-20.));
#40306=CARTESIAN_POINT('',(20.,47.5,-20.));
#40307=CARTESIAN_POINT('Origin',(20.,48.,-19.5));
#40308=CARTESIAN_POINT('',(0.,48.,-19.5));
#40309=CARTESIAN_POINT('',(0.,48.,-19.5));
#40310=CARTESIAN_POINT('',(20.,48.,-19.5));
#40311=CARTESIAN_POINT('',(20.,48.,-19.5));
#40312=CARTESIAN_POINT('',(20.,48.,-19.5));
#40313=CARTESIAN_POINT('Origin',(20.,48.,19.5));
#40314=CARTESIAN_POINT('',(0.,48.,19.5));
#40315=CARTESIAN_POINT('',(0.,48.,19.5));
#40316=CARTESIAN_POINT('',(20.,48.,19.5));
#40317=CARTESIAN_POINT('',(20.,48.,19.5));
#40318=CARTESIAN_POINT('',(20.,48.,19.5));
#40319=CARTESIAN_POINT('Origin',(20.,47.5,20.));
#40320=CARTESIAN_POINT('',(0.,47.5,20.));
#40321=CARTESIAN_POINT('',(0.,47.5,20.));
#40322=CARTESIAN_POINT('',(20.,47.5,20.));
#40323=CARTESIAN_POINT('',(20.,47.5,20.));
#40324=CARTESIAN_POINT('',(20.,47.5,20.));
#40325=CARTESIAN_POINT('Origin',(20.,47.5,20.));
#40326=CARTESIAN_POINT('',(0.,47.5,20.));
#40327=CARTESIAN_POINT('',(20.,47.5,20.));
#40328=CARTESIAN_POINT('Origin',(20.,0.,0.));
#40329=CARTESIAN_POINT('Origin',(0.,0.,0.));
#40330=CARTESIAN_POINT('Origin',(13.3,31.5,27.));
#40331=CARTESIAN_POINT('Origin',(13.3,31.5,-27.));
#40332=CARTESIAN_POINT('Origin',(5.5,44.,0.));
#40333=CARTESIAN_POINT('Origin',(14.5,35.5,0.));
#66657=UNCERTAINTY_MEASURE_WITH_UNIT(LENGTH_MEASURE(0.01),#66722,
'DISTANCE_ACCURACY_VALUE',
'Maximum model space distance between geometric entities at asserted c
onnectivities');
#66680=UNCERTAINTY_MEASURE_WITH_UNIT(LENGTH_MEASURE(0.01),#66722,
'DISTANCE_ACCURACY_VALUE',
'Maximum model space distance between geometric entities at asserted c
onnectivities');
#66698=(
GEOMETRIC_REPRESENTATION_CONTEXT(3)
GLOBAL_UNCERTAINTY_ASSIGNED_CONTEXT((#66657))
GLOBAL_UNIT_ASSIGNED_CONTEXT((#66722,#66724,#66725))
REPRESENTATION_CONTEXT('','3D')
);
#66721=(
GEOMETRIC_REPRESENTATION_CONTEXT(3)
GLOBAL_UNCERTAINTY_ASSIGNED_CONTEXT((#66680))
GLOBAL_UNIT_ASSIGNED_CONTEXT((#66722,#66724,#66725))
REPRESENTATION_CONTEXT('','3D')
);
#66722=(
LENGTH_UNIT()
NAMED_UNIT(*)
SI_UNIT(.MILLI.,.METRE.)
);
#66724=(
NAMED_UNIT(*)
PLANE_ANGLE_UNIT()
SI_UNIT($,.RADIAN.)
);
#66725=(
NAMED_UNIT(*)
SI_UNIT($,.STERADIAN.)
SOLID_ANGLE_UNIT()
);
#66743=SHAPE_DEFINITION_REPRESENTATION(#66797,#66907);
#66797=PRODUCT_DEFINITION_SHAPE('',$,#66948);
#66907=SHAPE_REPRESENTATION('',(#27395),#66698);
#66930=PRODUCT_DEFINITION_CONTEXT('part definition',#67052,'design');
#66948=PRODUCT_DEFINITION('Fixed Bearing Housing',
'Fixed Bearing Housing',#66988,#66930);
#66988=PRODUCT_DEFINITION_FORMATION('',$,#67071);
#67052=APPLICATION_CONTEXT(
'Core Data for Automotive Mechanical Design Process');
#67053=PRODUCT_CONTEXT('part definition',#67052,'mechanical');
#67071=PRODUCT('Fixed Bearing Housing','Fixed Bearing Housing',$,(#67053));
#67095=PRESENTATION_STYLE_ASSIGNMENT((#67097));
#67097=SURFACE_STYLE_USAGE(.BOTH.,#67099);
#67099=SURFACE_SIDE_STYLE('',(#67101));
#67101=SURFACE_STYLE_FILL_AREA(#67103);
#67103=FILL_AREA_STYLE('Opaque(202,209,238)',(#67105));
#67105=FILL_AREA_STYLE_COLOUR('Opaque(202,209,238)',#67107);
#67107=COLOUR_RGB('Opaque(202,209,238)',0.792156862745098,0.819607843137255,
0.933333333333333);
ENDSEC;
END-ISO-10303-21;
